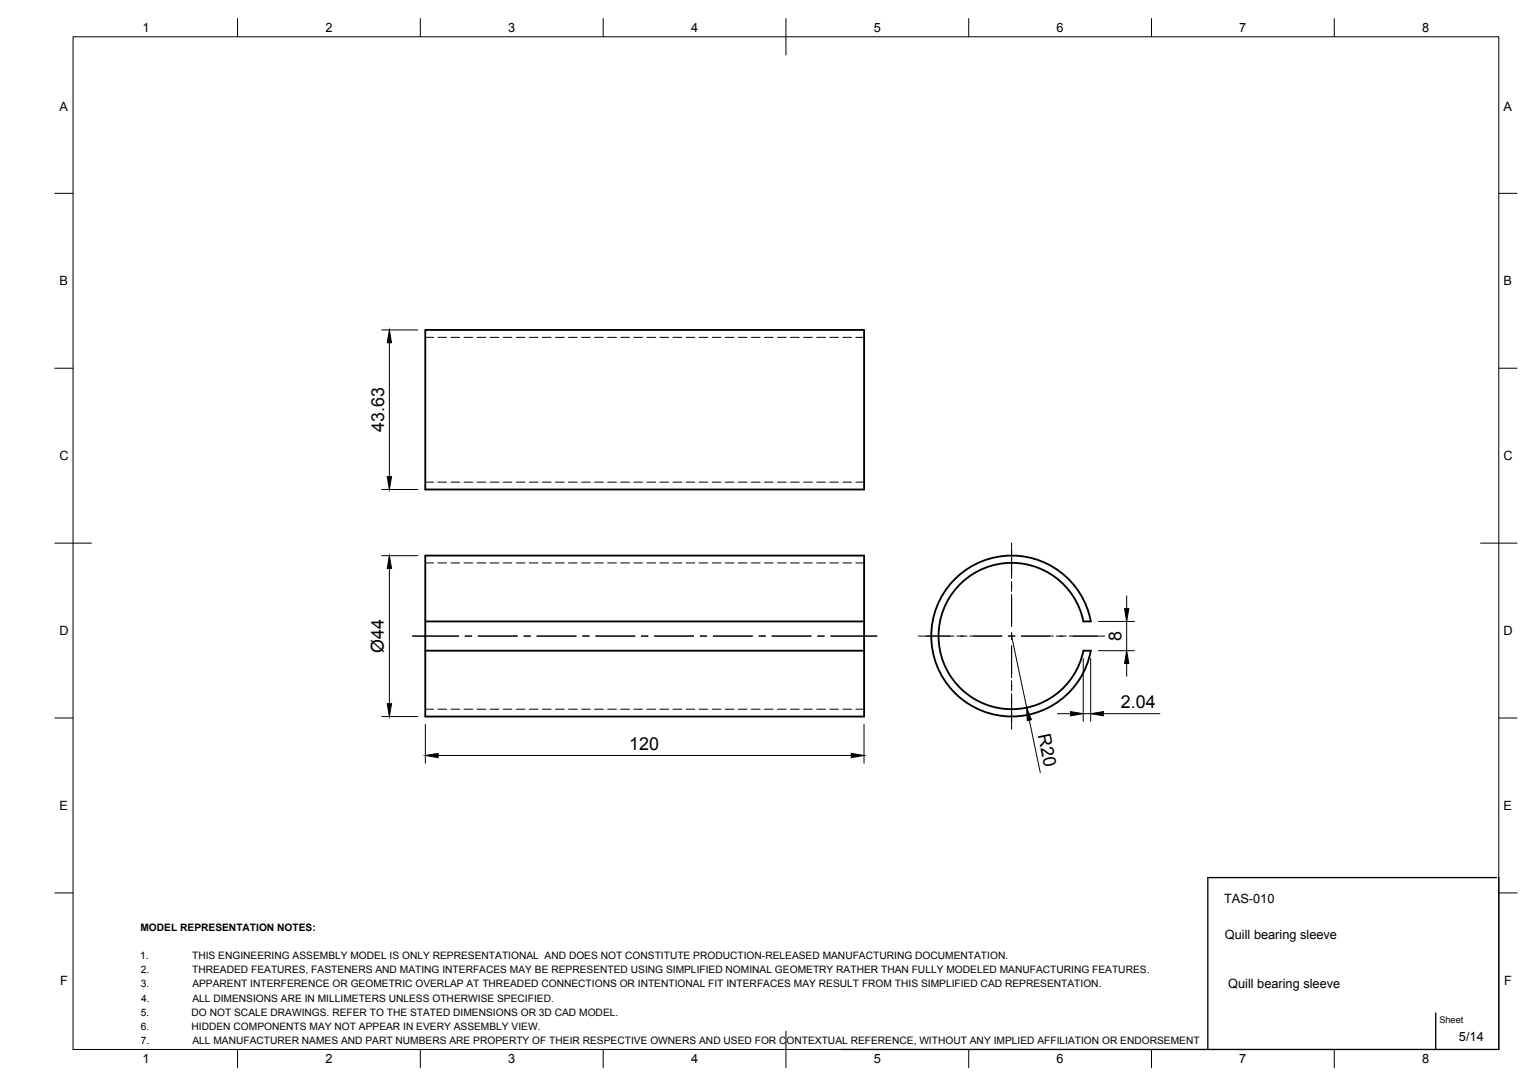
ISO-10303-21;
HEADER;
/* Generated by software containing ST-Developer
 * from STEP Tools, Inc. (www.steptools.com) 
 */

FILE_DESCRIPTION(
/* description */ (
'Independent keyed-quill tailstock, native coupled50mm slider andM16x2
 feed screw, conical dead center, bronze sleeves/thrust washers, cross
-pinned handwheel and bolted guide key. Custom center taper; no standa
rd taper compatibility, machine-bed compatibility or load rating assig
ned.'),
/* implementation_level */ '2;1');

FILE_NAME(
/* name */ 'Quill bearing sleeve.step',
/* time_stamp */ '2026-11-14T07:17:36-08:00',
/* author */ (''),
/* organization */ (''),
/* preprocessor_version */ 'ST-DEVELOPER v20.2',
/* originating_system */ 'Autodesk Translation Framework v15.17.0.0',
/* authorisation */ '');

FILE_SCHEMA (('AUTOMOTIVE_DESIGN { 1 0 10303 214 3 1 1 }'));
ENDSEC;

DATA;
#10=MECHANICAL_DESIGN_GEOMETRIC_PRESENTATION_REPRESENTATION('',(#155),#289387);
#121=SHAPE_REPRESENTATION_RELATIONSHIP('SRR','None',#289456,#138);
#138=ADVANCED_BREP_SHAPE_REPRESENTATION('',(#172),#289372);
#155=STYLED_ITEM('',(#289550),#172);
#172=MANIFOLD_SOLID_BREP('Body1',#16843);
#340=PLANE('',#17440);
#341=PLANE('',#17441);
#342=PLANE('',#17442);
#343=PLANE('',#17449);
#763=FACE_OUTER_BOUND('',#1444,.T.);
#764=FACE_OUTER_BOUND('',#1445,.T.);
#765=FACE_OUTER_BOUND('',#1446,.T.);
#766=FACE_OUTER_BOUND('',#1447,.T.);
#767=FACE_OUTER_BOUND('',#1448,.T.);
#768=FACE_OUTER_BOUND('',#1449,.T.);
#1444=EDGE_LOOP('',(#12915,#12916,#12917,#12918));
#1445=EDGE_LOOP('',(#12919,#12920,#12921,#12922));
#1446=EDGE_LOOP('',(#12923,#12924,#12925,#12926));
#1447=EDGE_LOOP('',(#12927,#12928,#12929,#12930));
#1448=EDGE_LOOP('',(#12931,#12932,#12933,#12934));
#1449=EDGE_LOOP('',(#12935,#12936,#12937,#12938));
#1879=CIRCLE('',#17443,22.);
#1880=CIRCLE('',#17444,20.);
#1881=CIRCLE('',#17446,20.);
#1882=CIRCLE('',#17448,22.);
#4256=LINE('',#136516,#4893);
#4257=LINE('',#136518,#4894);
#4258=LINE('',#136520,#4895);
#4259=LINE('',#136521,#4896);
#4260=LINE('',#136525,#4897);
#4261=LINE('',#136527,#4898);
#4262=LINE('',#136529,#4899);
#4263=LINE('',#136530,#4900);
#4893=VECTOR('',#18994,10.);
#4894=VECTOR('',#18995,10.);
#4895=VECTOR('',#18996,10.);
#4896=VECTOR('',#18997,10.);
#4897=VECTOR('',#19000,10.);
#4898=VECTOR('',#19001,10.);
#4899=VECTOR('',#19002,10.);
#4900=VECTOR('',#19003,10.);
#6267=VERTEX_POINT('',#136514);
#6268=VERTEX_POINT('',#136515);
#6269=VERTEX_POINT('',#136517);
#6270=VERTEX_POINT('',#136519);
#6271=VERTEX_POINT('',#136523);
#6272=VERTEX_POINT('',#136524);
#6273=VERTEX_POINT('',#136526);
#6274=VERTEX_POINT('',#136528);
#8769=EDGE_CURVE('',#6267,#6268,#4256,.T.);
#8770=EDGE_CURVE('',#6269,#6267,#4257,.T.);
#8771=EDGE_CURVE('',#6270,#6269,#4258,.T.);
#8772=EDGE_CURVE('',#6268,#6270,#4259,.T.);
#8773=EDGE_CURVE('',#6271,#6272,#4260,.T.);
#8774=EDGE_CURVE('',#6273,#6271,#4261,.T.);
#8775=EDGE_CURVE('',#6274,#6273,#4262,.T.);
#8776=EDGE_CURVE('',#6272,#6274,#4263,.T.);
#8777=EDGE_CURVE('',#6269,#6274,#1879,.T.);
#8778=EDGE_CURVE('',#6272,#6267,#1880,.T.);
#8779=EDGE_CURVE('',#6271,#6268,#1881,.T.);
#8780=EDGE_CURVE('',#6270,#6273,#1882,.T.);
#12915=ORIENTED_EDGE('',*,*,#8769,.F.);
#12916=ORIENTED_EDGE('',*,*,#8770,.F.);
#12917=ORIENTED_EDGE('',*,*,#8771,.F.);
#12918=ORIENTED_EDGE('',*,*,#8772,.F.);
#12919=ORIENTED_EDGE('',*,*,#8773,.F.);
#12920=ORIENTED_EDGE('',*,*,#8774,.F.);
#12921=ORIENTED_EDGE('',*,*,#8775,.F.);
#12922=ORIENTED_EDGE('',*,*,#8776,.F.);
#12923=ORIENTED_EDGE('',*,*,#8776,.T.);
#12924=ORIENTED_EDGE('',*,*,#8777,.F.);
#12925=ORIENTED_EDGE('',*,*,#8770,.T.);
#12926=ORIENTED_EDGE('',*,*,#8778,.F.);
#12927=ORIENTED_EDGE('',*,*,#8773,.T.);
#12928=ORIENTED_EDGE('',*,*,#8778,.T.);
#12929=ORIENTED_EDGE('',*,*,#8769,.T.);
#12930=ORIENTED_EDGE('',*,*,#8779,.F.);
#12931=ORIENTED_EDGE('',*,*,#8775,.T.);
#12932=ORIENTED_EDGE('',*,*,#8780,.F.);
#12933=ORIENTED_EDGE('',*,*,#8771,.T.);
#12934=ORIENTED_EDGE('',*,*,#8777,.T.);
#12935=ORIENTED_EDGE('',*,*,#8774,.T.);
#12936=ORIENTED_EDGE('',*,*,#8779,.T.);
#12937=ORIENTED_EDGE('',*,*,#8772,.T.);
#12938=ORIENTED_EDGE('',*,*,#8780,.T.);
#15982=CYLINDRICAL_SURFACE('',#17445,20.);
#15983=CYLINDRICAL_SURFACE('',#17447,22.);
#16531=ADVANCED_FACE('',(#763),#340,.F.);
#16532=ADVANCED_FACE('',(#764),#341,.F.);
#16533=ADVANCED_FACE('',(#765),#342,.F.);
#16534=ADVANCED_FACE('',(#766),#15982,.F.);
#16535=ADVANCED_FACE('',(#767),#15983,.T.);
#16536=ADVANCED_FACE('',(#768),#343,.T.);
#16843=CLOSED_SHELL('',(#16531,#16532,#16533,#16534,#16535,#16536));
#17439=AXIS2_PLACEMENT_3D('',#136512,#18990,#18991);
#17440=AXIS2_PLACEMENT_3D('',#136513,#18992,#18993);
#17441=AXIS2_PLACEMENT_3D('',#136522,#18998,#18999);
#17442=AXIS2_PLACEMENT_3D('',#136531,#19004,#19005);
#17443=AXIS2_PLACEMENT_3D('',#136532,#19006,#19007);
#17444=AXIS2_PLACEMENT_3D('',#136533,#19008,#19009);
#17445=AXIS2_PLACEMENT_3D('',#136534,#19010,#19011);
#17446=AXIS2_PLACEMENT_3D('',#136535,#19012,#19013);
#17447=AXIS2_PLACEMENT_3D('',#136536,#19014,#19015);
#17448=AXIS2_PLACEMENT_3D('',#136537,#19016,#19017);
#17449=AXIS2_PLACEMENT_3D('',#136538,#19018,#19019);
#18990=DIRECTION('axis',(0.,0.,1.));
#18991=DIRECTION('refdir',(1.,0.,0.));
#18992=DIRECTION('center_axis',(-1.,0.,0.));
#18993=DIRECTION('ref_axis',(0.,1.,0.));
#18994=DIRECTION('',(0.,0.,1.));
#18995=DIRECTION('',(0.,-1.,0.));
#18996=DIRECTION('',(0.,0.,-1.));
#18997=DIRECTION('',(0.,1.,0.));
#18998=DIRECTION('center_axis',(1.,0.,0.));
#18999=DIRECTION('ref_axis',(0.,-1.,0.));
#19000=DIRECTION('',(0.,0.,-1.));
#19001=DIRECTION('',(0.,-1.,0.));
#19002=DIRECTION('',(0.,0.,1.));
#19003=DIRECTION('',(0.,1.,0.));
#19004=DIRECTION('center_axis',(0.,0.,1.));
#19005=DIRECTION('ref_axis',(1.,0.,0.));
#19006=DIRECTION('center_axis',(0.,0.,1.));
#19007=DIRECTION('ref_axis',(1.,0.,0.));
#19008=DIRECTION('center_axis',(0.,0.,-1.));
#19009=DIRECTION('ref_axis',(1.,0.,0.));
#19010=DIRECTION('center_axis',(0.,0.,1.));
#19011=DIRECTION('ref_axis',(6.12323399573677E-17,-1.,0.));
#19012=DIRECTION('center_axis',(0.,0.,-1.));
#19013=DIRECTION('ref_axis',(1.,0.,0.));
#19014=DIRECTION('center_axis',(0.,0.,1.));
#19015=DIRECTION('ref_axis',(6.12323399573677E-17,-1.,0.));
#19016=DIRECTION('center_axis',(0.,0.,1.));
#19017=DIRECTION('ref_axis',(1.,0.,0.));
#19018=DIRECTION('center_axis',(0.,0.,1.));
#19019=DIRECTION('ref_axis',(1.,0.,0.));
#136512=CARTESIAN_POINT('',(0.,0.,0.));
#136513=CARTESIAN_POINT('Origin',(-4.,16.,120.));
#136514=CARTESIAN_POINT('',(-4.,19.5959179422654,0.));
#136515=CARTESIAN_POINT('',(-4.,19.5959179422654,120.));
#136516=CARTESIAN_POINT('',(-4.,19.5959179422654,0.));
#136517=CARTESIAN_POINT('',(-4.,21.6333076527839,0.));
#136518=CARTESIAN_POINT('',(-4.,8.,0.));
#136519=CARTESIAN_POINT('',(-4.,21.6333076527839,120.));
#136520=CARTESIAN_POINT('',(-4.,21.6333076527839,0.));
#136521=CARTESIAN_POINT('',(-4.,8.,120.));
#136522=CARTESIAN_POINT('Origin',(4.,24.,120.));
#136523=CARTESIAN_POINT('',(4.,19.5959179422654,120.));
#136524=CARTESIAN_POINT('',(4.,19.5959179422654,0.));
#136525=CARTESIAN_POINT('',(4.,19.5959179422654,0.));
#136526=CARTESIAN_POINT('',(4.,21.6333076527839,120.));
#136527=CARTESIAN_POINT('',(4.,12.,120.));
#136528=CARTESIAN_POINT('',(4.,21.6333076527839,0.));
#136529=CARTESIAN_POINT('',(4.,21.6333076527839,0.));
#136530=CARTESIAN_POINT('',(4.,12.,0.));
#136531=CARTESIAN_POINT('Origin',(0.,0.,0.));
#136532=CARTESIAN_POINT('Origin',(0.,0.,0.));
#136533=CARTESIAN_POINT('Origin',(0.,0.,0.));
#136534=CARTESIAN_POINT('Origin',(0.,0.,0.));
#136535=CARTESIAN_POINT('Origin',(0.,0.,120.));
#136536=CARTESIAN_POINT('Origin',(0.,0.,0.));
#136537=CARTESIAN_POINT('Origin',(0.,0.,120.));
#136538=CARTESIAN_POINT('Origin',(0.,0.,120.));
#289353=UNCERTAINTY_MEASURE_WITH_UNIT(LENGTH_MEASURE(0.01),#289388,
'DISTANCE_ACCURACY_VALUE',
'Maximum model space distance between geometric entities at asserted c
onnectivities');
#289368=UNCERTAINTY_MEASURE_WITH_UNIT(LENGTH_MEASURE(0.01),#289388,
'DISTANCE_ACCURACY_VALUE',
'Maximum model space distance between geometric entities at asserted c
onnectivities');
#289372=(
GEOMETRIC_REPRESENTATION_CONTEXT(3)
GLOBAL_UNCERTAINTY_ASSIGNED_CONTEXT((#289353))
GLOBAL_UNIT_ASSIGNED_CONTEXT((#289388,#289390,#289391))
REPRESENTATION_CONTEXT('','3D')
);
#289387=(
GEOMETRIC_REPRESENTATION_CONTEXT(3)
GLOBAL_UNCERTAINTY_ASSIGNED_CONTEXT((#289368))
GLOBAL_UNIT_ASSIGNED_CONTEXT((#289388,#289390,#289391))
REPRESENTATION_CONTEXT('','3D')
);
#289388=(
LENGTH_UNIT()
NAMED_UNIT(*)
SI_UNIT(.MILLI.,.METRE.)
);
#289390=(
NAMED_UNIT(*)
PLANE_ANGLE_UNIT()
SI_UNIT($,.RADIAN.)
);
#289391=(
NAMED_UNIT(*)
SI_UNIT($,.STERADIAN.)
SOLID_ANGLE_UNIT()
);
#289395=SHAPE_DEFINITION_REPRESENTATION(#289413,#289456);
#289413=PRODUCT_DEFINITION_SHAPE('',$,#289475);
#289456=SHAPE_REPRESENTATION('',(#17439),#289372);
#289471=PRODUCT_DEFINITION_CONTEXT('part definition',#289527,'design');
#289475=PRODUCT_DEFINITION('Quill bearing sleeve',
'Quill bearing sleeve',#289493,#289471);
#289493=PRODUCT_DEFINITION_FORMATION('',$,#289532);
#289527=APPLICATION_CONTEXT(
'Core Data for Automotive Mechanical Design Process');
#289528=PRODUCT_CONTEXT('part definition',#289527,'mechanical');
#289532=PRODUCT('Quill bearing sleeve','Quill bearing sleeve',$,(#289528));
#289550=PRESENTATION_STYLE_ASSIGNMENT((#289557));
#289557=SURFACE_STYLE_USAGE(.BOTH.,#289564);
#289564=SURFACE_SIDE_STYLE('',(#289571));
#289571=SURFACE_STYLE_FILL_AREA(#289578);
#289578=FILL_AREA_STYLE('Opaque(185,192,202)',(#289585));
#289585=FILL_AREA_STYLE_COLOUR('Opaque(185,192,202)',#289592);
#289592=COLOUR_RGB('Opaque(185,192,202)',0.725490196078431,0.752941176470588,
0.792156862745098);
ENDSEC;
END-ISO-10303-21;
